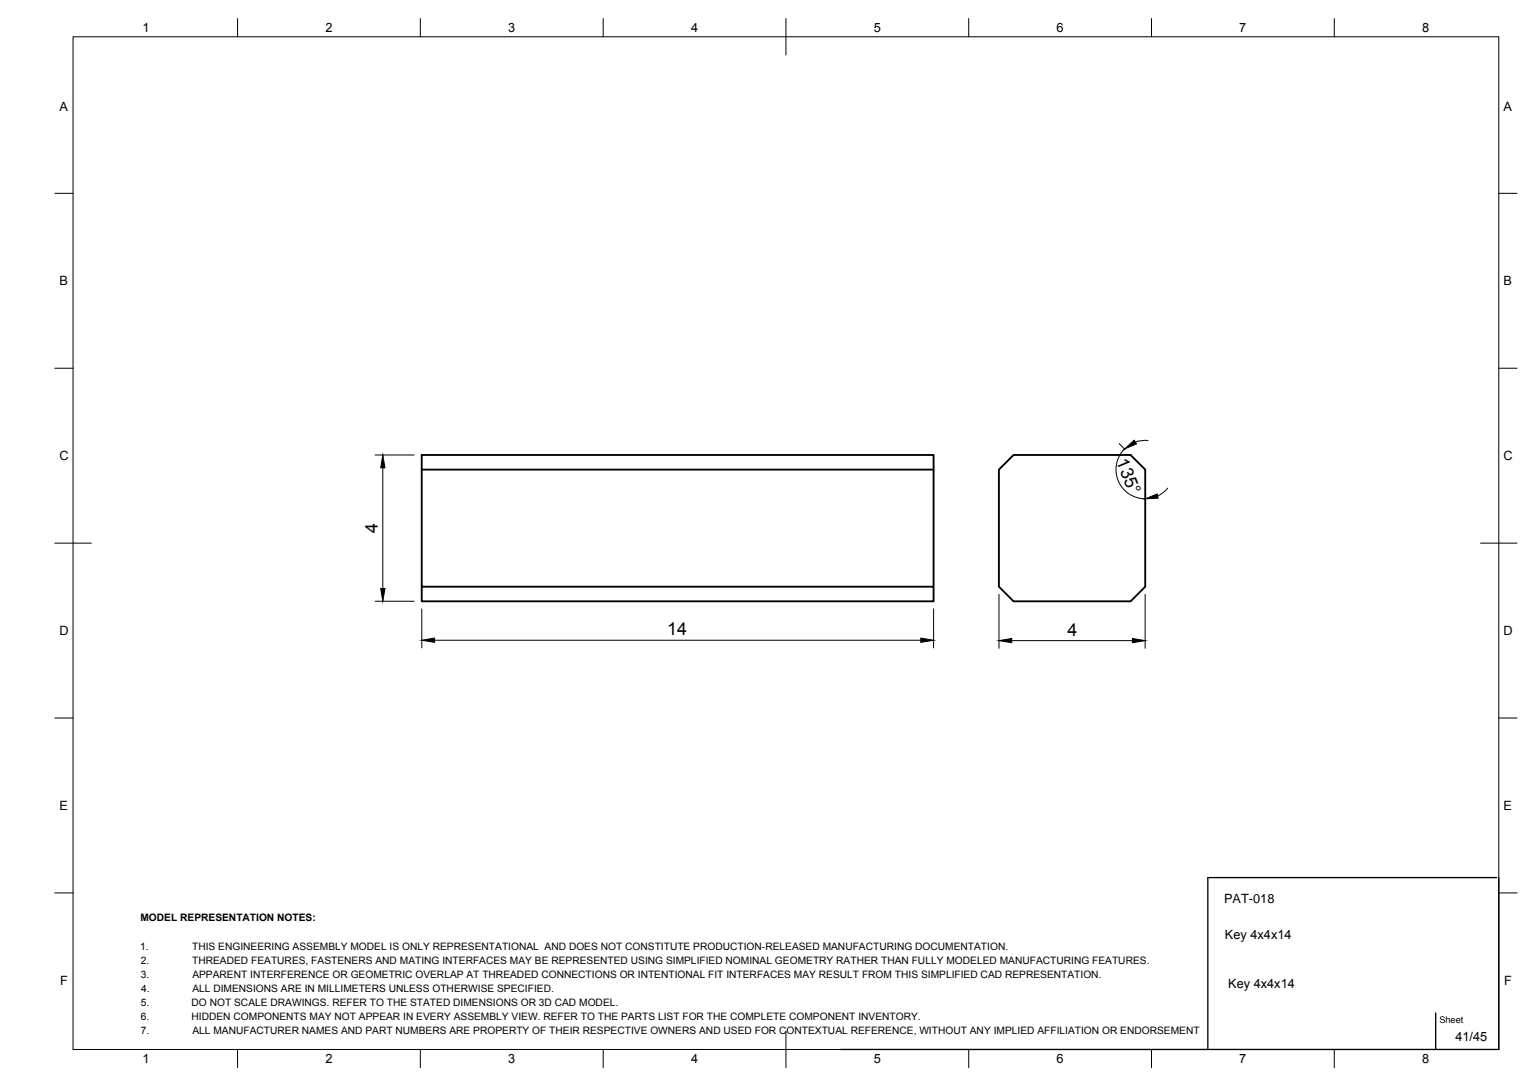
ISO-10303-21;
HEADER;
/* Generated by software containing ST-Developer
 * from STEP Tools, Inc. (www.steptools.com) 
 */

FILE_DESCRIPTION(
/* description */ ('Cam-driven reciprocating slide'),
/* implementation_level */ '2;1');

FILE_NAME(
/* name */ 'Key 4x4x14.step',
/* time_stamp */ '2026-10-28T03:25:20-07:00',
/* author */ (''),
/* organization */ (''),
/* preprocessor_version */ 'ST-DEVELOPER v20.2',
/* originating_system */ 'Autodesk Translation Framework v15.17.0.0',
/* authorisation */ '');

FILE_SCHEMA (('AUTOMOTIVE_DESIGN { 1 0 10303 214 3 1 1 }'));
ENDSEC;

DATA;
#10=MECHANICAL_DESIGN_GEOMETRIC_PRESENTATION_REPRESENTATION('',(#461),#13277);
#380=SHAPE_REPRESENTATION_RELATIONSHIP('SRR','None',#13476,#417);
#417=ADVANCED_BREP_SHAPE_REPRESENTATION('',(#503),#13271);
#461=STYLED_ITEM('',(#13720),#503);
#503=MANIFOLD_SOLID_BREP('Body1',#6439);
#864=PLANE('',#7522);
#865=PLANE('',#7523);
#866=PLANE('',#7524);
#867=PLANE('',#7525);
#868=PLANE('',#7526);
#869=PLANE('',#7527);
#870=PLANE('',#7528);
#871=PLANE('',#7529);
#872=PLANE('',#7530);
#873=PLANE('',#7531);
#1228=FACE_OUTER_BOUND('',#1766,.T.);
#1229=FACE_OUTER_BOUND('',#1767,.T.);
#1230=FACE_OUTER_BOUND('',#1768,.T.);
#1231=FACE_OUTER_BOUND('',#1769,.T.);
#1232=FACE_OUTER_BOUND('',#1770,.T.);
#1233=FACE_OUTER_BOUND('',#1771,.T.);
#1234=FACE_OUTER_BOUND('',#1772,.T.);
#1235=FACE_OUTER_BOUND('',#1773,.T.);
#1236=FACE_OUTER_BOUND('',#1774,.T.);
#1237=FACE_OUTER_BOUND('',#1775,.T.);
#1766=EDGE_LOOP('',(#5678,#5679,#5680,#5681,#5682,#5683,#5684,#5685));
#1767=EDGE_LOOP('',(#5686,#5687,#5688,#5689));
#1768=EDGE_LOOP('',(#5690,#5691,#5692,#5693));
#1769=EDGE_LOOP('',(#5694,#5695,#5696,#5697));
#1770=EDGE_LOOP('',(#5698,#5699,#5700,#5701));
#1771=EDGE_LOOP('',(#5702,#5703,#5704,#5705,#5706,#5707,#5708,#5709));
#1772=EDGE_LOOP('',(#5710,#5711,#5712,#5713));
#1773=EDGE_LOOP('',(#5714,#5715,#5716,#5717));
#1774=EDGE_LOOP('',(#5718,#5719,#5720,#5721));
#1775=EDGE_LOOP('',(#5722,#5723,#5724,#5725));
#2191=LINE('',#12895,#2630);
#2192=LINE('',#12897,#2631);
#2193=LINE('',#12899,#2632);
#2194=LINE('',#12901,#2633);
#2195=LINE('',#12903,#2634);
#2196=LINE('',#12905,#2635);
#2197=LINE('',#12907,#2636);
#2198=LINE('',#12908,#2637);
#2199=LINE('',#12911,#2638);
#2200=LINE('',#12913,#2639);
#2201=LINE('',#12914,#2640);
#2202=LINE('',#12917,#2641);
#2203=LINE('',#12918,#2642);
#2204=LINE('',#12921,#2643);
#2205=LINE('',#12922,#2644);
#2206=LINE('',#12925,#2645);
#2207=LINE('',#12926,#2646);
#2208=LINE('',#12929,#2647);
#2209=LINE('',#12931,#2648);
#2210=LINE('',#12933,#2649);
#2211=LINE('',#12934,#2650);
#2212=LINE('',#12936,#2651);
#2213=LINE('',#12938,#2652);
#2214=LINE('',#12940,#2653);
#2630=VECTOR('',#9367,1.);
#2631=VECTOR('',#9368,1.);
#2632=VECTOR('',#9369,1.);
#2633=VECTOR('',#9370,1.);
#2634=VECTOR('',#9371,1.);
#2635=VECTOR('',#9372,1.);
#2636=VECTOR('',#9373,1.);
#2637=VECTOR('',#9374,1.);
#2638=VECTOR('',#9377,1.);
#2639=VECTOR('',#9378,1.);
#2640=VECTOR('',#9379,1.);
#2641=VECTOR('',#9382,1.);
#2642=VECTOR('',#9383,1.);
#2643=VECTOR('',#9386,1.);
#2644=VECTOR('',#9387,1.);
#2645=VECTOR('',#9390,1.);
#2646=VECTOR('',#9391,1.);
#2647=VECTOR('',#9394,1.);
#2648=VECTOR('',#9395,1.);
#2649=VECTOR('',#9396,1.);
#2650=VECTOR('',#9397,1.);
#2651=VECTOR('',#9400,1.);
#2652=VECTOR('',#9403,1.);
#2653=VECTOR('',#9406,1.);
#3488=VERTEX_POINT('',#12893);
#3489=VERTEX_POINT('',#12894);
#3490=VERTEX_POINT('',#12896);
#3491=VERTEX_POINT('',#12898);
#3492=VERTEX_POINT('',#12900);
#3493=VERTEX_POINT('',#12902);
#3494=VERTEX_POINT('',#12904);
#3495=VERTEX_POINT('',#12906);
#3496=VERTEX_POINT('',#12910);
#3497=VERTEX_POINT('',#12912);
#3498=VERTEX_POINT('',#12916);
#3499=VERTEX_POINT('',#12920);
#3500=VERTEX_POINT('',#12924);
#3501=VERTEX_POINT('',#12928);
#3502=VERTEX_POINT('',#12930);
#3503=VERTEX_POINT('',#12932);
#4229=EDGE_CURVE('',#3488,#3489,#2191,.T.);
#4230=EDGE_CURVE('',#3490,#3488,#2192,.T.);
#4231=EDGE_CURVE('',#3491,#3490,#2193,.T.);
#4232=EDGE_CURVE('',#3492,#3491,#2194,.T.);
#4233=EDGE_CURVE('',#3493,#3492,#2195,.T.);
#4234=EDGE_CURVE('',#3494,#3493,#2196,.T.);
#4235=EDGE_CURVE('',#3495,#3494,#2197,.T.);
#4236=EDGE_CURVE('',#3489,#3495,#2198,.T.);
#4237=EDGE_CURVE('',#3492,#3496,#2199,.T.);
#4238=EDGE_CURVE('',#3496,#3497,#2200,.T.);
#4239=EDGE_CURVE('',#3497,#3493,#2201,.T.);
#4240=EDGE_CURVE('',#3498,#3491,#2202,.T.);
#4241=EDGE_CURVE('',#3498,#3496,#2203,.T.);
#4242=EDGE_CURVE('',#3490,#3499,#2204,.T.);
#4243=EDGE_CURVE('',#3499,#3498,#2205,.T.);
#4244=EDGE_CURVE('',#3500,#3488,#2206,.T.);
#4245=EDGE_CURVE('',#3500,#3499,#2207,.T.);
#4246=EDGE_CURVE('',#3501,#3500,#2208,.T.);
#4247=EDGE_CURVE('',#3502,#3501,#2209,.T.);
#4248=EDGE_CURVE('',#3503,#3502,#2210,.T.);
#4249=EDGE_CURVE('',#3497,#3503,#2211,.T.);
#4250=EDGE_CURVE('',#3489,#3501,#2212,.T.);
#4251=EDGE_CURVE('',#3502,#3495,#2213,.T.);
#4252=EDGE_CURVE('',#3494,#3503,#2214,.T.);
#5678=ORIENTED_EDGE('',*,*,#4229,.F.);
#5679=ORIENTED_EDGE('',*,*,#4230,.F.);
#5680=ORIENTED_EDGE('',*,*,#4231,.F.);
#5681=ORIENTED_EDGE('',*,*,#4232,.F.);
#5682=ORIENTED_EDGE('',*,*,#4233,.F.);
#5683=ORIENTED_EDGE('',*,*,#4234,.F.);
#5684=ORIENTED_EDGE('',*,*,#4235,.F.);
#5685=ORIENTED_EDGE('',*,*,#4236,.F.);
#5686=ORIENTED_EDGE('',*,*,#4233,.T.);
#5687=ORIENTED_EDGE('',*,*,#4237,.T.);
#5688=ORIENTED_EDGE('',*,*,#4238,.T.);
#5689=ORIENTED_EDGE('',*,*,#4239,.T.);
#5690=ORIENTED_EDGE('',*,*,#4232,.T.);
#5691=ORIENTED_EDGE('',*,*,#4240,.F.);
#5692=ORIENTED_EDGE('',*,*,#4241,.T.);
#5693=ORIENTED_EDGE('',*,*,#4237,.F.);
#5694=ORIENTED_EDGE('',*,*,#4231,.T.);
#5695=ORIENTED_EDGE('',*,*,#4242,.T.);
#5696=ORIENTED_EDGE('',*,*,#4243,.T.);
#5697=ORIENTED_EDGE('',*,*,#4240,.T.);
#5698=ORIENTED_EDGE('',*,*,#4230,.T.);
#5699=ORIENTED_EDGE('',*,*,#4244,.F.);
#5700=ORIENTED_EDGE('',*,*,#4245,.T.);
#5701=ORIENTED_EDGE('',*,*,#4242,.F.);
#5702=ORIENTED_EDGE('',*,*,#4238,.F.);
#5703=ORIENTED_EDGE('',*,*,#4241,.F.);
#5704=ORIENTED_EDGE('',*,*,#4243,.F.);
#5705=ORIENTED_EDGE('',*,*,#4245,.F.);
#5706=ORIENTED_EDGE('',*,*,#4246,.F.);
#5707=ORIENTED_EDGE('',*,*,#4247,.F.);
#5708=ORIENTED_EDGE('',*,*,#4248,.F.);
#5709=ORIENTED_EDGE('',*,*,#4249,.F.);
#5710=ORIENTED_EDGE('',*,*,#4229,.T.);
#5711=ORIENTED_EDGE('',*,*,#4250,.T.);
#5712=ORIENTED_EDGE('',*,*,#4246,.T.);
#5713=ORIENTED_EDGE('',*,*,#4244,.T.);
#5714=ORIENTED_EDGE('',*,*,#4236,.T.);
#5715=ORIENTED_EDGE('',*,*,#4251,.F.);
#5716=ORIENTED_EDGE('',*,*,#4247,.T.);
#5717=ORIENTED_EDGE('',*,*,#4250,.F.);
#5718=ORIENTED_EDGE('',*,*,#4235,.T.);
#5719=ORIENTED_EDGE('',*,*,#4252,.T.);
#5720=ORIENTED_EDGE('',*,*,#4248,.T.);
#5721=ORIENTED_EDGE('',*,*,#4251,.T.);
#5722=ORIENTED_EDGE('',*,*,#4234,.T.);
#5723=ORIENTED_EDGE('',*,*,#4239,.F.);
#5724=ORIENTED_EDGE('',*,*,#4249,.T.);
#5725=ORIENTED_EDGE('',*,*,#4252,.F.);
#6346=ADVANCED_FACE('',(#1228),#864,.T.);
#6347=ADVANCED_FACE('',(#1229),#865,.T.);
#6348=ADVANCED_FACE('',(#1230),#866,.T.);
#6349=ADVANCED_FACE('',(#1231),#867,.T.);
#6350=ADVANCED_FACE('',(#1232),#868,.T.);
#6351=ADVANCED_FACE('',(#1233),#869,.F.);
#6352=ADVANCED_FACE('',(#1234),#870,.T.);
#6353=ADVANCED_FACE('',(#1235),#871,.T.);
#6354=ADVANCED_FACE('',(#1236),#872,.T.);
#6355=ADVANCED_FACE('',(#1237),#873,.F.);
#6439=CLOSED_SHELL('',(#6346,#6347,#6348,#6349,#6350,#6351,#6352,#6353,
#6354,#6355));
#7521=AXIS2_PLACEMENT_3D('',#12891,#9363,#9364);
#7522=AXIS2_PLACEMENT_3D('',#12892,#9365,#9366);
#7523=AXIS2_PLACEMENT_3D('',#12909,#9375,#9376);
#7524=AXIS2_PLACEMENT_3D('',#12915,#9380,#9381);
#7525=AXIS2_PLACEMENT_3D('',#12919,#9384,#9385);
#7526=AXIS2_PLACEMENT_3D('',#12923,#9388,#9389);
#7527=AXIS2_PLACEMENT_3D('',#12927,#9392,#9393);
#7528=AXIS2_PLACEMENT_3D('',#12935,#9398,#9399);
#7529=AXIS2_PLACEMENT_3D('',#12937,#9401,#9402);
#7530=AXIS2_PLACEMENT_3D('',#12939,#9404,#9405);
#7531=AXIS2_PLACEMENT_3D('',#12941,#9407,#9408);
#9363=DIRECTION('axis',(0.,0.,1.));
#9364=DIRECTION('refdir',(1.,0.,0.));
#9365=DIRECTION('center_axis',(1.,0.,0.));
#9366=DIRECTION('ref_axis',(0.,0.,-1.));
#9367=DIRECTION('',(0.,0.707106781186547,-0.707106781186548));
#9368=DIRECTION('',(0.,1.,0.));
#9369=DIRECTION('',(0.,0.707106781186547,0.707106781186548));
#9370=DIRECTION('',(0.,0.,1.));
#9371=DIRECTION('',(0.,-0.707106781186548,0.707106781186548));
#9372=DIRECTION('',(0.,-1.,0.));
#9373=DIRECTION('',(0.,-0.707106781186548,-0.707106781186548));
#9374=DIRECTION('',(0.,0.,-1.));
#9375=DIRECTION('center_axis',(0.,-0.707106781186548,-0.707106781186548));
#9376=DIRECTION('ref_axis',(-1.,0.,0.));
#9377=DIRECTION('',(-1.,0.,0.));
#9378=DIRECTION('',(0.,0.707106781186548,-0.707106781186548));
#9379=DIRECTION('',(1.,0.,0.));
#9380=DIRECTION('center_axis',(0.,-1.,0.));
#9381=DIRECTION('ref_axis',(1.,0.,0.));
#9382=DIRECTION('',(1.,0.,0.));
#9383=DIRECTION('',(0.,0.,-1.));
#9384=DIRECTION('center_axis',(0.,-0.707106781186548,0.707106781186547));
#9385=DIRECTION('ref_axis',(1.,0.,0.));
#9386=DIRECTION('',(-1.,0.,0.));
#9387=DIRECTION('',(0.,-0.707106781186547,-0.707106781186548));
#9388=DIRECTION('center_axis',(0.,0.,1.));
#9389=DIRECTION('ref_axis',(1.,0.,0.));
#9390=DIRECTION('',(1.,0.,0.));
#9391=DIRECTION('',(0.,-1.,0.));
#9392=DIRECTION('center_axis',(1.,0.,0.));
#9393=DIRECTION('ref_axis',(0.,0.,-1.));
#9394=DIRECTION('',(0.,-0.707106781186547,0.707106781186548));
#9395=DIRECTION('',(0.,0.,1.));
#9396=DIRECTION('',(0.,0.707106781186548,0.707106781186548));
#9397=DIRECTION('',(0.,1.,0.));
#9398=DIRECTION('center_axis',(0.,0.707106781186548,0.707106781186547));
#9399=DIRECTION('ref_axis',(1.,0.,0.));
#9400=DIRECTION('',(-1.,0.,0.));
#9401=DIRECTION('center_axis',(0.,1.,0.));
#9402=DIRECTION('ref_axis',(-1.,0.,0.));
#9403=DIRECTION('',(1.,0.,0.));
#9404=DIRECTION('center_axis',(0.,0.707106781186548,-0.707106781186548));
#9405=DIRECTION('ref_axis',(-1.,0.,0.));
#9406=DIRECTION('',(-1.,0.,0.));
#9407=DIRECTION('center_axis',(0.,0.,1.));
#9408=DIRECTION('ref_axis',(1.,0.,0.));
#12891=CARTESIAN_POINT('',(0.,0.,0.));
#12892=CARTESIAN_POINT('Origin',(0.7,0.,0.25));
#12893=CARTESIAN_POINT('',(0.7,0.16,0.4));
#12894=CARTESIAN_POINT('',(0.7,0.2,0.36));
#12895=CARTESIAN_POINT('',(0.7,0.1675,0.3925));
#12896=CARTESIAN_POINT('',(0.7,-0.16,0.4));
#12897=CARTESIAN_POINT('',(0.7,0.,0.4));
#12898=CARTESIAN_POINT('',(0.7,-0.2,0.36));
#12899=CARTESIAN_POINT('',(0.7,-0.1675,0.3925));
#12900=CARTESIAN_POINT('',(0.7,-0.2,0.04));
#12901=CARTESIAN_POINT('',(0.7,-0.2,0.125));
#12902=CARTESIAN_POINT('',(0.7,-0.16,0.));
#12903=CARTESIAN_POINT('',(0.7,-0.1925,0.0325));
#12904=CARTESIAN_POINT('',(0.7,0.16,0.));
#12905=CARTESIAN_POINT('',(0.7,0.,0.));
#12906=CARTESIAN_POINT('',(0.7,0.2,0.04));
#12907=CARTESIAN_POINT('',(0.7,0.1925,0.0325));
#12908=CARTESIAN_POINT('',(0.7,0.2,0.125));
#12909=CARTESIAN_POINT('Origin',(-0.4,-0.18,0.02));
#12910=CARTESIAN_POINT('',(-0.7,-0.2,0.04));
#12911=CARTESIAN_POINT('',(-0.4,-0.2,0.04));
#12912=CARTESIAN_POINT('',(-0.7,-0.16,0.));
#12913=CARTESIAN_POINT('',(-0.7,-0.1925,0.0325));
#12914=CARTESIAN_POINT('',(-0.4,-0.16,0.));
#12915=CARTESIAN_POINT('Origin',(-0.8,-0.2,0.));
#12916=CARTESIAN_POINT('',(-0.7,-0.2,0.36));
#12917=CARTESIAN_POINT('',(-0.4,-0.2,0.36));
#12918=CARTESIAN_POINT('',(-0.7,-0.2,0.125));
#12919=CARTESIAN_POINT('Origin',(-0.4,-0.18,0.38));
#12920=CARTESIAN_POINT('',(-0.7,-0.16,0.4));
#12921=CARTESIAN_POINT('',(-0.4,-0.16,0.4));
#12922=CARTESIAN_POINT('',(-0.7,-0.1675,0.3925));
#12923=CARTESIAN_POINT('Origin',(0.,0.,0.4));
#12924=CARTESIAN_POINT('',(-0.7,0.16,0.4));
#12925=CARTESIAN_POINT('',(0.4,0.16,0.4));
#12926=CARTESIAN_POINT('',(-0.7,0.,0.4));
#12927=CARTESIAN_POINT('Origin',(-0.7,0.,0.25));
#12928=CARTESIAN_POINT('',(-0.7,0.2,0.36));
#12929=CARTESIAN_POINT('',(-0.7,0.1675,0.3925));
#12930=CARTESIAN_POINT('',(-0.7,0.2,0.04));
#12931=CARTESIAN_POINT('',(-0.7,0.2,0.125));
#12932=CARTESIAN_POINT('',(-0.7,0.16,0.));
#12933=CARTESIAN_POINT('',(-0.7,0.1925,0.0325));
#12934=CARTESIAN_POINT('',(-0.7,0.,0.));
#12935=CARTESIAN_POINT('Origin',(0.4,0.18,0.38));
#12936=CARTESIAN_POINT('',(0.4,0.2,0.36));
#12937=CARTESIAN_POINT('Origin',(0.8,0.2,0.));
#12938=CARTESIAN_POINT('',(0.4,0.2,0.04));
#12939=CARTESIAN_POINT('Origin',(0.4,0.18,0.02));
#12940=CARTESIAN_POINT('',(0.4,0.16,0.));
#12941=CARTESIAN_POINT('Origin',(0.,0.,0.));
#13227=UNCERTAINTY_MEASURE_WITH_UNIT(LENGTH_MEASURE(0.001),#13278,
'DISTANCE_ACCURACY_VALUE',
'Maximum model space distance between geometric entities at asserted c
onnectivities');
#13233=UNCERTAINTY_MEASURE_WITH_UNIT(LENGTH_MEASURE(0.001),#13278,
'DISTANCE_ACCURACY_VALUE',
'Maximum model space distance between geometric entities at asserted c
onnectivities');
#13271=(
GEOMETRIC_REPRESENTATION_CONTEXT(3)
GLOBAL_UNCERTAINTY_ASSIGNED_CONTEXT((#13227))
GLOBAL_UNIT_ASSIGNED_CONTEXT((#13278,#13280,#13281))
REPRESENTATION_CONTEXT('','3D')
);
#13277=(
GEOMETRIC_REPRESENTATION_CONTEXT(3)
GLOBAL_UNCERTAINTY_ASSIGNED_CONTEXT((#13233))
GLOBAL_UNIT_ASSIGNED_CONTEXT((#13278,#13280,#13281))
REPRESENTATION_CONTEXT('','3D')
);
#13278=(
LENGTH_UNIT()
NAMED_UNIT(*)
SI_UNIT(.CENTI.,.METRE.)
);
#13280=(
NAMED_UNIT(*)
PLANE_ANGLE_UNIT()
SI_UNIT($,.RADIAN.)
);
#13281=(
NAMED_UNIT(*)
SI_UNIT($,.STERADIAN.)
SOLID_ANGLE_UNIT()
);
#13319=SHAPE_DEFINITION_REPRESENTATION(#13369,#13476);
#13369=PRODUCT_DEFINITION_SHAPE('',$,#13520);
#13476=SHAPE_REPRESENTATION('',(#7521),#13271);
#13482=PRODUCT_DEFINITION_CONTEXT('part definition',#13613,'design');
#13520=PRODUCT_DEFINITION('Key 4x4x14','Key 4x4x14',#13563,#13482);
#13563=PRODUCT_DEFINITION_FORMATION('',$,#13652);
#13613=APPLICATION_CONTEXT(
'Core Data for Automotive Mechanical Design Process');
#13614=PRODUCT_CONTEXT('part definition',#13613,'mechanical');
#13652=PRODUCT('Key 4x4x14','Key 4x4x14','Key 4x4x14',(#13614));
#13714=COLOUR_RGB('Grey',0.48,0.52,0.57);
#13715=FILL_AREA_STYLE_COLOUR('',#13714);
#13716=FILL_AREA_STYLE('',(#13715));
#13717=SURFACE_STYLE_FILL_AREA(#13716);
#13718=SURFACE_SIDE_STYLE('',(#13717));
#13719=SURFACE_STYLE_USAGE(.BOTH.,#13718);
#13720=PRESENTATION_STYLE_ASSIGNMENT((#13719));
ENDSEC;
END-ISO-10303-21;
